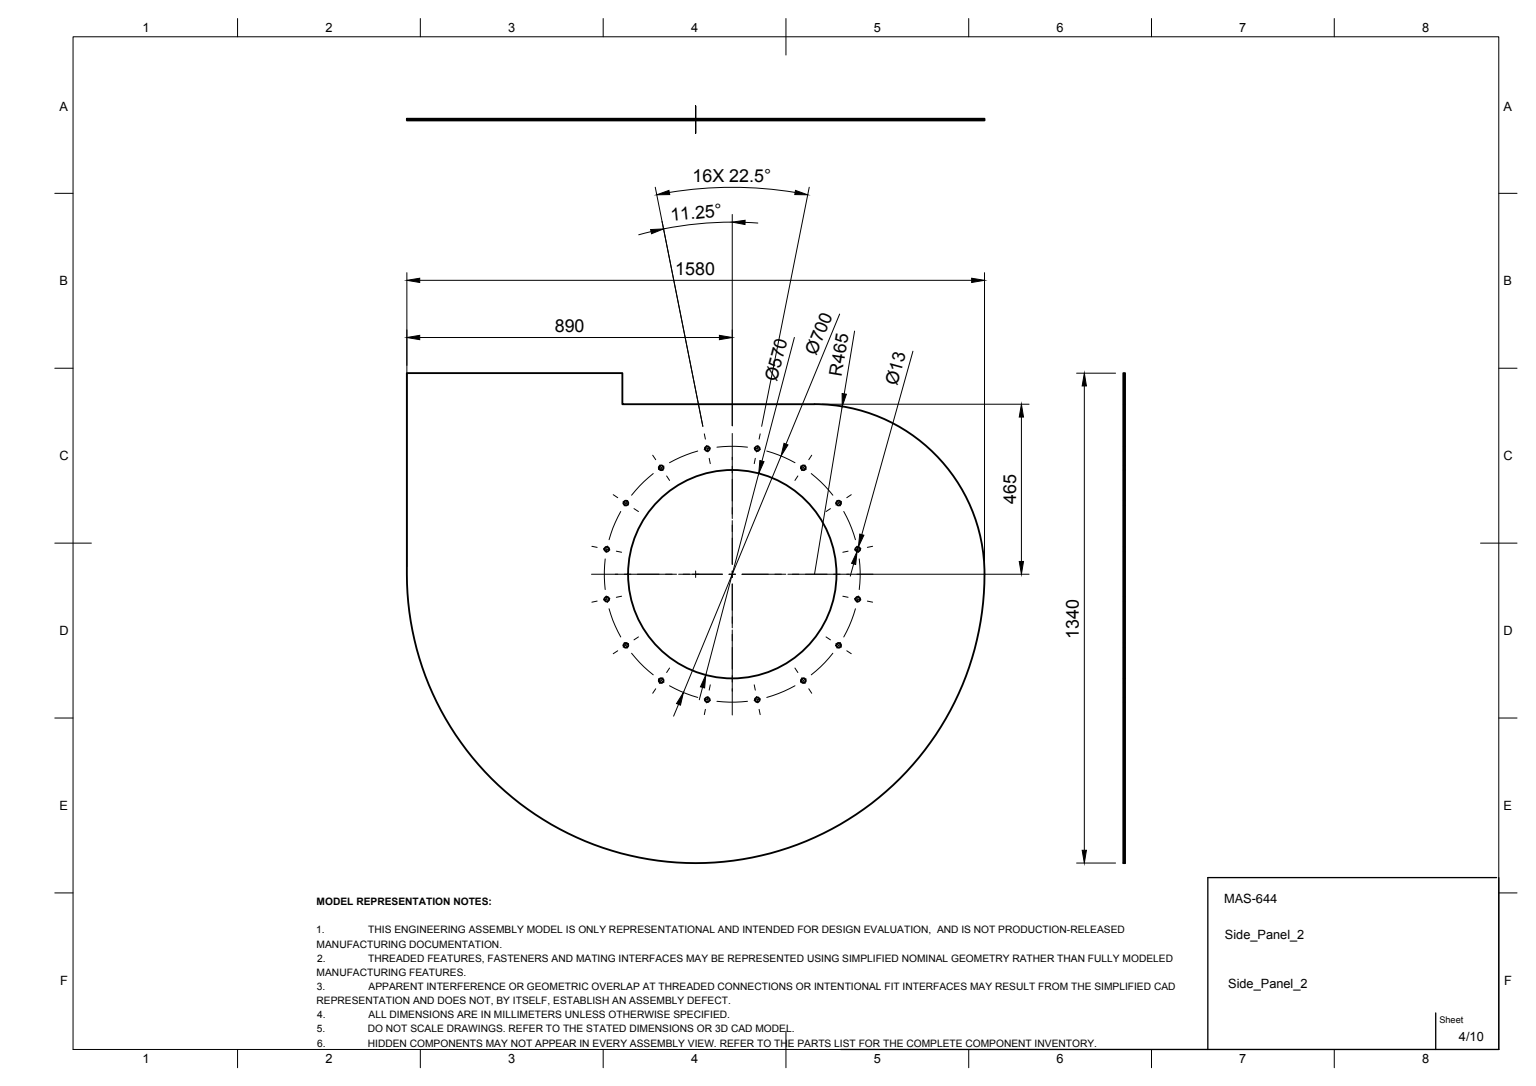
ISO-10303-21;
HEADER;
FILE_DESCRIPTION((''),'2;1');
FILE_NAME('Side_Panel_2.step','2026-10-09T11:38:21-07:00',(''),(''),'','','');
FILE_SCHEMA (('AUTOMOTIVE_DESIGN { 1 0 10303 214 3 1 1 }'));
ENDSEC;
DATA;
#10=MECHANICAL_DESIGN_GEOMETRIC_PRESENTATION_REPRESENTATION('',(#60),#3619);
#44=SHAPE_REPRESENTATION_RELATIONSHIP('SRR','None',#3652,#52) ;
#52=ADVANCED_BREP_SHAPE_REPRESENTATION('',(#68),#3612) ;
#60=STYLED_ITEM('',(#3700),#68) ;
#68=MANIFOLD_SOLID_BREP('Body1',#2084) ;
#77=FACE_BOUND('',#356,.T.) ;
#78=FACE_BOUND('',#357,.T.) ;
#79=FACE_BOUND('',#358,.T.) ;
#80=FACE_BOUND('',#359,.T.) ;
#81=FACE_BOUND('',#360,.T.) ;
#82=FACE_BOUND('',#361,.T.) ;
#83=FACE_BOUND('',#362,.T.) ;
#84=FACE_BOUND('',#363,.T.) ;
#85=FACE_BOUND('',#364,.T.) ;
#86=FACE_BOUND('',#365,.T.) ;
#87=FACE_BOUND('',#366,.T.) ;
#88=FACE_BOUND('',#367,.T.) ;
#89=FACE_BOUND('',#368,.T.) ;
#90=FACE_BOUND('',#369,.T.) ;
#91=FACE_BOUND('',#370,.T.) ;
#92=FACE_BOUND('',#371,.T.) ;
#93=FACE_BOUND('',#372,.T.) ;
#94=FACE_BOUND('',#374,.T.) ;
#95=FACE_BOUND('',#375,.T.) ;
#96=FACE_BOUND('',#376,.T.) ;
#97=FACE_BOUND('',#377,.T.) ;
#98=FACE_BOUND('',#378,.T.) ;
#99=FACE_BOUND('',#379,.T.) ;
#100=FACE_BOUND('',#380,.T.) ;
#101=FACE_BOUND('',#381,.T.) ;
#102=FACE_BOUND('',#382,.T.) ;
#103=FACE_BOUND('',#383,.T.) ;
#104=FACE_BOUND('',#384,.T.) ;
#105=FACE_BOUND('',#385,.T.) ;
#106=FACE_BOUND('',#386,.T.) ;
#107=FACE_BOUND('',#387,.T.) ;
#108=FACE_BOUND('',#388,.T.) ;
#109=FACE_BOUND('',#389,.T.) ;
#110=FACE_BOUND('',#390,.T.) ;
#163=PLANE('',#2249) ;
#164=PLANE('',#2250) ;
#165=PLANE('',#2251) ;
#166=PLANE('',#2252) ;
#167=PLANE('',#2259) ;
#168=PLANE('',#2260) ;
#222=FACE_OUTER_BOUND('',#332,.T.) ;
#223=FACE_OUTER_BOUND('',#333,.T.) ;
#224=FACE_OUTER_BOUND('',#334,.T.) ;
#225=FACE_OUTER_BOUND('',#335,.T.) ;
#226=FACE_OUTER_BOUND('',#336,.T.) ;
#227=FACE_OUTER_BOUND('',#337,.T.) ;
#228=FACE_OUTER_BOUND('',#338,.T.) ;
#229=FACE_OUTER_BOUND('',#339,.T.) ;
#230=FACE_OUTER_BOUND('',#340,.T.) ;
#231=FACE_OUTER_BOUND('',#341,.T.) ;
#232=FACE_OUTER_BOUND('',#342,.T.) ;
#233=FACE_OUTER_BOUND('',#343,.T.) ;
#234=FACE_OUTER_BOUND('',#344,.T.) ;
#235=FACE_OUTER_BOUND('',#345,.T.) ;
#236=FACE_OUTER_BOUND('',#346,.T.) ;
#237=FACE_OUTER_BOUND('',#347,.T.) ;
#238=FACE_OUTER_BOUND('',#348,.T.) ;
#239=FACE_OUTER_BOUND('',#349,.T.) ;
#240=FACE_OUTER_BOUND('',#350,.T.) ;
#241=FACE_OUTER_BOUND('',#351,.T.) ;
#242=FACE_OUTER_BOUND('',#352,.T.) ;
#243=FACE_OUTER_BOUND('',#353,.T.) ;
#244=FACE_OUTER_BOUND('',#354,.T.) ;
#245=FACE_OUTER_BOUND('',#355,.T.) ;
#246=FACE_OUTER_BOUND('',#373,.T.) ;
#332=EDGE_LOOP('',(#1429,#1430,#1431,#1432)) ;
#333=EDGE_LOOP('',(#1433,#1434,#1435,#1436)) ;
#334=EDGE_LOOP('',(#1437,#1438,#1439,#1440)) ;
#335=EDGE_LOOP('',(#1441,#1442,#1443,#1444)) ;
#336=EDGE_LOOP('',(#1445,#1446,#1447,#1448)) ;
#337=EDGE_LOOP('',(#1449,#1450,#1451,#1452)) ;
#338=EDGE_LOOP('',(#1453,#1454,#1455,#1456)) ;
#339=EDGE_LOOP('',(#1457,#1458,#1459,#1460)) ;
#340=EDGE_LOOP('',(#1461,#1462,#1463,#1464)) ;
#341=EDGE_LOOP('',(#1465,#1466,#1467,#1468)) ;
#342=EDGE_LOOP('',(#1469,#1470,#1471,#1472)) ;
#343=EDGE_LOOP('',(#1473,#1474,#1475,#1476)) ;
#344=EDGE_LOOP('',(#1477,#1478,#1479,#1480)) ;
#345=EDGE_LOOP('',(#1481,#1482,#1483,#1484)) ;
#346=EDGE_LOOP('',(#1485,#1486,#1487,#1488)) ;
#347=EDGE_LOOP('',(#1489,#1490,#1491,#1492)) ;
#348=EDGE_LOOP('',(#1493,#1494,#1495,#1496)) ;
#349=EDGE_LOOP('',(#1497,#1498,#1499,#1500)) ;
#350=EDGE_LOOP('',(#1501,#1502,#1503,#1504)) ;
#351=EDGE_LOOP('',(#1505,#1506,#1507,#1508)) ;
#352=EDGE_LOOP('',(#1509,#1510,#1511,#1512)) ;
#353=EDGE_LOOP('',(#1513,#1514,#1515,#1516)) ;
#354=EDGE_LOOP('',(#1517,#1518,#1519,#1520)) ;
#355=EDGE_LOOP('',(#1521,#1522,#1523,#1524,#1525,#1526)) ;
#356=EDGE_LOOP('',(#1527)) ;
#357=EDGE_LOOP('',(#1528)) ;
#358=EDGE_LOOP('',(#1529)) ;
#359=EDGE_LOOP('',(#1530)) ;
#360=EDGE_LOOP('',(#1531)) ;
#361=EDGE_LOOP('',(#1532)) ;
#362=EDGE_LOOP('',(#1533)) ;
#363=EDGE_LOOP('',(#1534)) ;
#364=EDGE_LOOP('',(#1535)) ;
#365=EDGE_LOOP('',(#1536)) ;
#366=EDGE_LOOP('',(#1537)) ;
#367=EDGE_LOOP('',(#1538)) ;
#368=EDGE_LOOP('',(#1539)) ;
#369=EDGE_LOOP('',(#1540)) ;
#370=EDGE_LOOP('',(#1541)) ;
#371=EDGE_LOOP('',(#1542)) ;
#372=EDGE_LOOP('',(#1543)) ;
#373=EDGE_LOOP('',(#1544,#1545,#1546,#1547,#1548,#1549)) ;
#374=EDGE_LOOP('',(#1550)) ;
#375=EDGE_LOOP('',(#1551)) ;
#376=EDGE_LOOP('',(#1552)) ;
#377=EDGE_LOOP('',(#1553)) ;
#378=EDGE_LOOP('',(#1554)) ;
#379=EDGE_LOOP('',(#1555)) ;
#380=EDGE_LOOP('',(#1556)) ;
#381=EDGE_LOOP('',(#1557)) ;
#382=EDGE_LOOP('',(#1558)) ;
#383=EDGE_LOOP('',(#1559)) ;
#384=EDGE_LOOP('',(#1560)) ;
#385=EDGE_LOOP('',(#1561)) ;
#386=EDGE_LOOP('',(#1562)) ;
#387=EDGE_LOOP('',(#1563)) ;
#388=EDGE_LOOP('',(#1564)) ;
#389=EDGE_LOOP('',(#1565)) ;
#390=EDGE_LOOP('',(#1566)) ;
#526=LINE('',#3082,#690) ;
#527=LINE('',#3088,#691) ;
#528=LINE('',#3094,#692) ;
#529=LINE('',#3100,#693) ;
#530=LINE('',#3106,#694) ;
#531=LINE('',#3112,#695) ;
#532=LINE('',#3118,#696) ;
#533=LINE('',#3124,#697) ;
#534=LINE('',#3130,#698) ;
#535=LINE('',#3136,#699) ;
#536=LINE('',#3142,#700) ;
#537=LINE('',#3148,#701) ;
#538=LINE('',#3154,#702) ;
#539=LINE('',#3160,#703) ;
#540=LINE('',#3166,#704) ;
#541=LINE('',#3172,#705) ;
#542=LINE('',#3178,#706) ;
#543=LINE('',#3183,#707) ;
#544=LINE('',#3185,#708) ;
#545=LINE('',#3187,#709) ;
#546=LINE('',#3188,#710) ;
#547=LINE('',#3191,#711) ;
#548=LINE('',#3193,#712) ;
#549=LINE('',#3194,#713) ;
#550=LINE('',#3197,#714) ;
#551=LINE('',#3199,#715) ;
#552=LINE('',#3200,#716) ;
#553=LINE('',#3203,#717) ;
#554=LINE('',#3205,#718) ;
#555=LINE('',#3206,#719) ;
#556=LINE('',#3211,#720) ;
#690=VECTOR('',#2464,6.50000000001752) ;
#691=VECTOR('',#2471,6.50000000000472) ;
#692=VECTOR('',#2478,6.50000000000422) ;
#693=VECTOR('',#2485,6.50000000000406) ;
#694=VECTOR('',#2492,6.50000000000367) ;
#695=VECTOR('',#2499,6.50000000000261) ;
#696=VECTOR('',#2506,6.50000000000162) ;
#697=VECTOR('',#2513,6.50000000000089) ;
#698=VECTOR('',#2520,6.50000000000024) ;
#699=VECTOR('',#2527,6.49999999999945) ;
#700=VECTOR('',#2534,6.49999999999912) ;
#701=VECTOR('',#2541,6.49999999999901) ;
#702=VECTOR('',#2548,6.49999999999912) ;
#703=VECTOR('',#2555,6.49999999999928) ;
#704=VECTOR('',#2562,6.4999999999921) ;
#705=VECTOR('',#2569,6.50000000000001) ;
#706=VECTOR('',#2576,285.) ;
#707=VECTOR('',#2581,1000.) ;
#708=VECTOR('',#2582,1000.) ;
#709=VECTOR('',#2583,1000.) ;
#710=VECTOR('',#2584,1000.) ;
#711=VECTOR('',#2587,1000.) ;
#712=VECTOR('',#2588,1000.) ;
#713=VECTOR('',#2589,1000.) ;
#714=VECTOR('',#2592,1000.) ;
#715=VECTOR('',#2593,1000.) ;
#716=VECTOR('',#2594,1000.) ;
#717=VECTOR('',#2597,1000.) ;
#718=VECTOR('',#2598,1000.) ;
#719=VECTOR('',#2599,1000.) ;
#720=VECTOR('',#2604,1000.) ;
#845=CIRCLE('',#2199,6.50000000001752) ;
#846=CIRCLE('',#2200,6.50000000001752) ;
#847=CIRCLE('',#2202,6.50000000000472) ;
#848=CIRCLE('',#2203,6.50000000000472) ;
#849=CIRCLE('',#2205,6.50000000000422) ;
#850=CIRCLE('',#2206,6.50000000000422) ;
#851=CIRCLE('',#2208,6.50000000000406) ;
#852=CIRCLE('',#2209,6.50000000000406) ;
#853=CIRCLE('',#2211,6.50000000000367) ;
#854=CIRCLE('',#2212,6.50000000000367) ;
#855=CIRCLE('',#2214,6.50000000000261) ;
#856=CIRCLE('',#2215,6.50000000000261) ;
#857=CIRCLE('',#2217,6.50000000000162) ;
#858=CIRCLE('',#2218,6.50000000000162) ;
#859=CIRCLE('',#2220,6.50000000000089) ;
#860=CIRCLE('',#2221,6.50000000000089) ;
#861=CIRCLE('',#2223,6.50000000000024) ;
#862=CIRCLE('',#2224,6.50000000000024) ;
#863=CIRCLE('',#2226,6.49999999999945) ;
#864=CIRCLE('',#2227,6.49999999999945) ;
#865=CIRCLE('',#2229,6.49999999999912) ;
#866=CIRCLE('',#2230,6.49999999999912) ;
#867=CIRCLE('',#2232,6.49999999999901) ;
#868=CIRCLE('',#2233,6.49999999999901) ;
#869=CIRCLE('',#2235,6.49999999999912) ;
#870=CIRCLE('',#2236,6.49999999999912) ;
#871=CIRCLE('',#2238,6.49999999999928) ;
#872=CIRCLE('',#2239,6.49999999999928) ;
#873=CIRCLE('',#2241,6.4999999999921) ;
#874=CIRCLE('',#2242,6.4999999999921) ;
#875=CIRCLE('',#2244,6.50000000000001) ;
#876=CIRCLE('',#2245,6.50000000000001) ;
#877=CIRCLE('',#2247,285.) ;
#878=CIRCLE('',#2248,285.) ;
#879=CIRCLE('',#2254,790.) ;
#880=CIRCLE('',#2255,790.) ;
#881=CIRCLE('',#2257,465.) ;
#882=CIRCLE('',#2258,465.) ;
#957=VERTEX_POINT('',#3079) ;
#958=VERTEX_POINT('',#3081) ;
#959=VERTEX_POINT('',#3085) ;
#960=VERTEX_POINT('',#3087) ;
#961=VERTEX_POINT('',#3091) ;
#962=VERTEX_POINT('',#3093) ;
#963=VERTEX_POINT('',#3097) ;
#964=VERTEX_POINT('',#3099) ;
#965=VERTEX_POINT('',#3103) ;
#966=VERTEX_POINT('',#3105) ;
#967=VERTEX_POINT('',#3109) ;
#968=VERTEX_POINT('',#3111) ;
#969=VERTEX_POINT('',#3115) ;
#970=VERTEX_POINT('',#3117) ;
#971=VERTEX_POINT('',#3121) ;
#972=VERTEX_POINT('',#3123) ;
#973=VERTEX_POINT('',#3127) ;
#974=VERTEX_POINT('',#3129) ;
#975=VERTEX_POINT('',#3133) ;
#976=VERTEX_POINT('',#3135) ;
#977=VERTEX_POINT('',#3139) ;
#978=VERTEX_POINT('',#3141) ;
#979=VERTEX_POINT('',#3145) ;
#980=VERTEX_POINT('',#3147) ;
#981=VERTEX_POINT('',#3151) ;
#982=VERTEX_POINT('',#3153) ;
#983=VERTEX_POINT('',#3157) ;
#984=VERTEX_POINT('',#3159) ;
#985=VERTEX_POINT('',#3163) ;
#986=VERTEX_POINT('',#3165) ;
#987=VERTEX_POINT('',#3169) ;
#988=VERTEX_POINT('',#3171) ;
#989=VERTEX_POINT('',#3175) ;
#990=VERTEX_POINT('',#3177) ;
#991=VERTEX_POINT('',#3181) ;
#992=VERTEX_POINT('',#3182) ;
#993=VERTEX_POINT('',#3184) ;
#994=VERTEX_POINT('',#3186) ;
#995=VERTEX_POINT('',#3190) ;
#996=VERTEX_POINT('',#3192) ;
#997=VERTEX_POINT('',#3196) ;
#998=VERTEX_POINT('',#3198) ;
#999=VERTEX_POINT('',#3202) ;
#1000=VERTEX_POINT('',#3204) ;
#1001=VERTEX_POINT('',#3208) ;
#1002=VERTEX_POINT('',#3210) ;
#1140=EDGE_CURVE('',#957,#957,#845,.T.) ;
#1141=EDGE_CURVE('',#957,#958,#526,.T.) ;
#1142=EDGE_CURVE('',#958,#958,#846,.T.) ;
#1143=EDGE_CURVE('',#959,#959,#847,.T.) ;
#1144=EDGE_CURVE('',#959,#960,#527,.T.) ;
#1145=EDGE_CURVE('',#960,#960,#848,.T.) ;
#1146=EDGE_CURVE('',#961,#961,#849,.T.) ;
#1147=EDGE_CURVE('',#961,#962,#528,.T.) ;
#1148=EDGE_CURVE('',#962,#962,#850,.T.) ;
#1149=EDGE_CURVE('',#963,#963,#851,.T.) ;
#1150=EDGE_CURVE('',#963,#964,#529,.T.) ;
#1151=EDGE_CURVE('',#964,#964,#852,.T.) ;
#1152=EDGE_CURVE('',#965,#965,#853,.T.) ;
#1153=EDGE_CURVE('',#965,#966,#530,.T.) ;
#1154=EDGE_CURVE('',#966,#966,#854,.T.) ;
#1155=EDGE_CURVE('',#967,#967,#855,.T.) ;
#1156=EDGE_CURVE('',#967,#968,#531,.T.) ;
#1157=EDGE_CURVE('',#968,#968,#856,.T.) ;
#1158=EDGE_CURVE('',#969,#969,#857,.T.) ;
#1159=EDGE_CURVE('',#969,#970,#532,.T.) ;
#1160=EDGE_CURVE('',#970,#970,#858,.T.) ;
#1161=EDGE_CURVE('',#971,#971,#859,.T.) ;
#1162=EDGE_CURVE('',#971,#972,#533,.T.) ;
#1163=EDGE_CURVE('',#972,#972,#860,.T.) ;
#1164=EDGE_CURVE('',#973,#973,#861,.T.) ;
#1165=EDGE_CURVE('',#973,#974,#534,.T.) ;
#1166=EDGE_CURVE('',#974,#974,#862,.T.) ;
#1167=EDGE_CURVE('',#975,#975,#863,.T.) ;
#1168=EDGE_CURVE('',#975,#976,#535,.T.) ;
#1169=EDGE_CURVE('',#976,#976,#864,.T.) ;
#1170=EDGE_CURVE('',#977,#977,#865,.T.) ;
#1171=EDGE_CURVE('',#977,#978,#536,.T.) ;
#1172=EDGE_CURVE('',#978,#978,#866,.T.) ;
#1173=EDGE_CURVE('',#979,#979,#867,.T.) ;
#1174=EDGE_CURVE('',#979,#980,#537,.T.) ;
#1175=EDGE_CURVE('',#980,#980,#868,.T.) ;
#1176=EDGE_CURVE('',#981,#981,#869,.T.) ;
#1177=EDGE_CURVE('',#981,#982,#538,.T.) ;
#1178=EDGE_CURVE('',#982,#982,#870,.T.) ;
#1179=EDGE_CURVE('',#983,#983,#871,.T.) ;
#1180=EDGE_CURVE('',#983,#984,#539,.T.) ;
#1181=EDGE_CURVE('',#984,#984,#872,.T.) ;
#1182=EDGE_CURVE('',#985,#985,#873,.T.) ;
#1183=EDGE_CURVE('',#985,#986,#540,.T.) ;
#1184=EDGE_CURVE('',#986,#986,#874,.T.) ;
#1185=EDGE_CURVE('',#987,#987,#875,.T.) ;
#1186=EDGE_CURVE('',#987,#988,#541,.T.) ;
#1187=EDGE_CURVE('',#988,#988,#876,.T.) ;
#1188=EDGE_CURVE('',#989,#989,#877,.T.) ;
#1189=EDGE_CURVE('',#989,#990,#542,.T.) ;
#1190=EDGE_CURVE('',#990,#990,#878,.T.) ;
#1191=EDGE_CURVE('',#991,#992,#543,.T.) ;
#1192=EDGE_CURVE('',#993,#991,#544,.T.) ;
#1193=EDGE_CURVE('',#993,#994,#545,.T.) ;
#1194=EDGE_CURVE('',#994,#992,#546,.T.) ;
#1195=EDGE_CURVE('',#995,#991,#547,.T.) ;
#1196=EDGE_CURVE('',#996,#995,#548,.T.) ;
#1197=EDGE_CURVE('',#996,#993,#549,.T.) ;
#1198=EDGE_CURVE('',#997,#995,#550,.T.) ;
#1199=EDGE_CURVE('',#998,#997,#551,.T.) ;
#1200=EDGE_CURVE('',#998,#996,#552,.T.) ;
#1201=EDGE_CURVE('',#999,#997,#553,.T.) ;
#1202=EDGE_CURVE('',#1000,#999,#554,.T.) ;
#1203=EDGE_CURVE('',#1000,#998,#555,.T.) ;
#1204=EDGE_CURVE('',#1001,#999,#879,.T.) ;
#1205=EDGE_CURVE('',#1002,#1001,#556,.T.) ;
#1206=EDGE_CURVE('',#1002,#1000,#880,.T.) ;
#1207=EDGE_CURVE('',#992,#1001,#881,.T.) ;
#1208=EDGE_CURVE('',#994,#1002,#882,.T.) ;
#1429=ORIENTED_EDGE('',*,*,#1140,.F.) ;
#1430=ORIENTED_EDGE('',*,*,#1141,.T.) ;
#1431=ORIENTED_EDGE('',*,*,#1142,.T.) ;
#1432=ORIENTED_EDGE('',*,*,#1141,.F.) ;
#1433=ORIENTED_EDGE('',*,*,#1143,.F.) ;
#1434=ORIENTED_EDGE('',*,*,#1144,.T.) ;
#1435=ORIENTED_EDGE('',*,*,#1145,.T.) ;
#1436=ORIENTED_EDGE('',*,*,#1144,.F.) ;
#1437=ORIENTED_EDGE('',*,*,#1146,.F.) ;
#1438=ORIENTED_EDGE('',*,*,#1147,.T.) ;
#1439=ORIENTED_EDGE('',*,*,#1148,.T.) ;
#1440=ORIENTED_EDGE('',*,*,#1147,.F.) ;
#1441=ORIENTED_EDGE('',*,*,#1149,.F.) ;
#1442=ORIENTED_EDGE('',*,*,#1150,.T.) ;
#1443=ORIENTED_EDGE('',*,*,#1151,.T.) ;
#1444=ORIENTED_EDGE('',*,*,#1150,.F.) ;
#1445=ORIENTED_EDGE('',*,*,#1152,.F.) ;
#1446=ORIENTED_EDGE('',*,*,#1153,.T.) ;
#1447=ORIENTED_EDGE('',*,*,#1154,.T.) ;
#1448=ORIENTED_EDGE('',*,*,#1153,.F.) ;
#1449=ORIENTED_EDGE('',*,*,#1155,.F.) ;
#1450=ORIENTED_EDGE('',*,*,#1156,.T.) ;
#1451=ORIENTED_EDGE('',*,*,#1157,.T.) ;
#1452=ORIENTED_EDGE('',*,*,#1156,.F.) ;
#1453=ORIENTED_EDGE('',*,*,#1158,.F.) ;
#1454=ORIENTED_EDGE('',*,*,#1159,.T.) ;
#1455=ORIENTED_EDGE('',*,*,#1160,.T.) ;
#1456=ORIENTED_EDGE('',*,*,#1159,.F.) ;
#1457=ORIENTED_EDGE('',*,*,#1161,.F.) ;
#1458=ORIENTED_EDGE('',*,*,#1162,.T.) ;
#1459=ORIENTED_EDGE('',*,*,#1163,.T.) ;
#1460=ORIENTED_EDGE('',*,*,#1162,.F.) ;
#1461=ORIENTED_EDGE('',*,*,#1164,.F.) ;
#1462=ORIENTED_EDGE('',*,*,#1165,.T.) ;
#1463=ORIENTED_EDGE('',*,*,#1166,.T.) ;
#1464=ORIENTED_EDGE('',*,*,#1165,.F.) ;
#1465=ORIENTED_EDGE('',*,*,#1167,.F.) ;
#1466=ORIENTED_EDGE('',*,*,#1168,.T.) ;
#1467=ORIENTED_EDGE('',*,*,#1169,.T.) ;
#1468=ORIENTED_EDGE('',*,*,#1168,.F.) ;
#1469=ORIENTED_EDGE('',*,*,#1170,.F.) ;
#1470=ORIENTED_EDGE('',*,*,#1171,.T.) ;
#1471=ORIENTED_EDGE('',*,*,#1172,.T.) ;
#1472=ORIENTED_EDGE('',*,*,#1171,.F.) ;
#1473=ORIENTED_EDGE('',*,*,#1173,.F.) ;
#1474=ORIENTED_EDGE('',*,*,#1174,.T.) ;
#1475=ORIENTED_EDGE('',*,*,#1175,.T.) ;
#1476=ORIENTED_EDGE('',*,*,#1174,.F.) ;
#1477=ORIENTED_EDGE('',*,*,#1176,.F.) ;
#1478=ORIENTED_EDGE('',*,*,#1177,.T.) ;
#1479=ORIENTED_EDGE('',*,*,#1178,.T.) ;
#1480=ORIENTED_EDGE('',*,*,#1177,.F.) ;
#1481=ORIENTED_EDGE('',*,*,#1179,.F.) ;
#1482=ORIENTED_EDGE('',*,*,#1180,.T.) ;
#1483=ORIENTED_EDGE('',*,*,#1181,.T.) ;
#1484=ORIENTED_EDGE('',*,*,#1180,.F.) ;
#1485=ORIENTED_EDGE('',*,*,#1182,.F.) ;
#1486=ORIENTED_EDGE('',*,*,#1183,.T.) ;
#1487=ORIENTED_EDGE('',*,*,#1184,.T.) ;
#1488=ORIENTED_EDGE('',*,*,#1183,.F.) ;
#1489=ORIENTED_EDGE('',*,*,#1185,.F.) ;
#1490=ORIENTED_EDGE('',*,*,#1186,.T.) ;
#1491=ORIENTED_EDGE('',*,*,#1187,.T.) ;
#1492=ORIENTED_EDGE('',*,*,#1186,.F.) ;
#1493=ORIENTED_EDGE('',*,*,#1188,.F.) ;
#1494=ORIENTED_EDGE('',*,*,#1189,.T.) ;
#1495=ORIENTED_EDGE('',*,*,#1190,.T.) ;
#1496=ORIENTED_EDGE('',*,*,#1189,.F.) ;
#1497=ORIENTED_EDGE('',*,*,#1191,.F.) ;
#1498=ORIENTED_EDGE('',*,*,#1192,.F.) ;
#1499=ORIENTED_EDGE('',*,*,#1193,.T.) ;
#1500=ORIENTED_EDGE('',*,*,#1194,.T.) ;
#1501=ORIENTED_EDGE('',*,*,#1195,.F.) ;
#1502=ORIENTED_EDGE('',*,*,#1196,.F.) ;
#1503=ORIENTED_EDGE('',*,*,#1197,.T.) ;
#1504=ORIENTED_EDGE('',*,*,#1192,.T.) ;
#1505=ORIENTED_EDGE('',*,*,#1198,.F.) ;
#1506=ORIENTED_EDGE('',*,*,#1199,.F.) ;
#1507=ORIENTED_EDGE('',*,*,#1200,.T.) ;
#1508=ORIENTED_EDGE('',*,*,#1196,.T.) ;
#1509=ORIENTED_EDGE('',*,*,#1201,.F.) ;
#1510=ORIENTED_EDGE('',*,*,#1202,.F.) ;
#1511=ORIENTED_EDGE('',*,*,#1203,.T.) ;
#1512=ORIENTED_EDGE('',*,*,#1199,.T.) ;
#1513=ORIENTED_EDGE('',*,*,#1204,.F.) ;
#1514=ORIENTED_EDGE('',*,*,#1205,.F.) ;
#1515=ORIENTED_EDGE('',*,*,#1206,.T.) ;
#1516=ORIENTED_EDGE('',*,*,#1202,.T.) ;
#1517=ORIENTED_EDGE('',*,*,#1207,.F.) ;
#1518=ORIENTED_EDGE('',*,*,#1194,.F.) ;
#1519=ORIENTED_EDGE('',*,*,#1208,.T.) ;
#1520=ORIENTED_EDGE('',*,*,#1205,.T.) ;
#1521=ORIENTED_EDGE('',*,*,#1193,.F.) ;
#1522=ORIENTED_EDGE('',*,*,#1197,.F.) ;
#1523=ORIENTED_EDGE('',*,*,#1200,.F.) ;
#1524=ORIENTED_EDGE('',*,*,#1203,.F.) ;
#1525=ORIENTED_EDGE('',*,*,#1206,.F.) ;
#1526=ORIENTED_EDGE('',*,*,#1208,.F.) ;
#1527=ORIENTED_EDGE('',*,*,#1140,.T.) ;
#1528=ORIENTED_EDGE('',*,*,#1143,.T.) ;
#1529=ORIENTED_EDGE('',*,*,#1146,.T.) ;
#1530=ORIENTED_EDGE('',*,*,#1149,.T.) ;
#1531=ORIENTED_EDGE('',*,*,#1152,.T.) ;
#1532=ORIENTED_EDGE('',*,*,#1155,.T.) ;
#1533=ORIENTED_EDGE('',*,*,#1158,.T.) ;
#1534=ORIENTED_EDGE('',*,*,#1161,.T.) ;
#1535=ORIENTED_EDGE('',*,*,#1164,.T.) ;
#1536=ORIENTED_EDGE('',*,*,#1167,.T.) ;
#1537=ORIENTED_EDGE('',*,*,#1170,.T.) ;
#1538=ORIENTED_EDGE('',*,*,#1173,.T.) ;
#1539=ORIENTED_EDGE('',*,*,#1176,.T.) ;
#1540=ORIENTED_EDGE('',*,*,#1179,.T.) ;
#1541=ORIENTED_EDGE('',*,*,#1182,.T.) ;
#1542=ORIENTED_EDGE('',*,*,#1185,.T.) ;
#1543=ORIENTED_EDGE('',*,*,#1188,.T.) ;
#1544=ORIENTED_EDGE('',*,*,#1191,.T.) ;
#1545=ORIENTED_EDGE('',*,*,#1207,.T.) ;
#1546=ORIENTED_EDGE('',*,*,#1204,.T.) ;
#1547=ORIENTED_EDGE('',*,*,#1201,.T.) ;
#1548=ORIENTED_EDGE('',*,*,#1198,.T.) ;
#1549=ORIENTED_EDGE('',*,*,#1195,.T.) ;
#1550=ORIENTED_EDGE('',*,*,#1142,.F.) ;
#1551=ORIENTED_EDGE('',*,*,#1145,.F.) ;
#1552=ORIENTED_EDGE('',*,*,#1148,.F.) ;
#1553=ORIENTED_EDGE('',*,*,#1151,.F.) ;
#1554=ORIENTED_EDGE('',*,*,#1154,.F.) ;
#1555=ORIENTED_EDGE('',*,*,#1157,.F.) ;
#1556=ORIENTED_EDGE('',*,*,#1160,.F.) ;
#1557=ORIENTED_EDGE('',*,*,#1163,.F.) ;
#1558=ORIENTED_EDGE('',*,*,#1166,.F.) ;
#1559=ORIENTED_EDGE('',*,*,#1169,.F.) ;
#1560=ORIENTED_EDGE('',*,*,#1172,.F.) ;
#1561=ORIENTED_EDGE('',*,*,#1175,.F.) ;
#1562=ORIENTED_EDGE('',*,*,#1178,.F.) ;
#1563=ORIENTED_EDGE('',*,*,#1181,.F.) ;
#1564=ORIENTED_EDGE('',*,*,#1184,.F.) ;
#1565=ORIENTED_EDGE('',*,*,#1187,.F.) ;
#1566=ORIENTED_EDGE('',*,*,#1190,.F.) ;
#1926=CYLINDRICAL_SURFACE('',#2198,6.50000000001752) ;
#1927=CYLINDRICAL_SURFACE('',#2201,6.50000000000472) ;
#1928=CYLINDRICAL_SURFACE('',#2204,6.50000000000422) ;
#1929=CYLINDRICAL_SURFACE('',#2207,6.50000000000406) ;
#1930=CYLINDRICAL_SURFACE('',#2210,6.50000000000367) ;
#1931=CYLINDRICAL_SURFACE('',#2213,6.50000000000261) ;
#1932=CYLINDRICAL_SURFACE('',#2216,6.50000000000162) ;
#1933=CYLINDRICAL_SURFACE('',#2219,6.50000000000089) ;
#1934=CYLINDRICAL_SURFACE('',#2222,6.50000000000024) ;
#1935=CYLINDRICAL_SURFACE('',#2225,6.49999999999945) ;
#1936=CYLINDRICAL_SURFACE('',#2228,6.49999999999912) ;
#1937=CYLINDRICAL_SURFACE('',#2231,6.49999999999901) ;
#1938=CYLINDRICAL_SURFACE('',#2234,6.49999999999912) ;
#1939=CYLINDRICAL_SURFACE('',#2237,6.49999999999928) ;
#1940=CYLINDRICAL_SURFACE('',#2240,6.4999999999921) ;
#1941=CYLINDRICAL_SURFACE('',#2243,6.50000000000001) ;
#1942=CYLINDRICAL_SURFACE('',#2246,285.) ;
#1943=CYLINDRICAL_SURFACE('',#2253,790.) ;
#1944=CYLINDRICAL_SURFACE('',#2256,465.) ;
#1984=ADVANCED_FACE('',(#222),#1926,.F.) ;
#1985=ADVANCED_FACE('',(#223),#1927,.F.) ;
#1986=ADVANCED_FACE('',(#224),#1928,.F.) ;
#1987=ADVANCED_FACE('',(#225),#1929,.F.) ;
#1988=ADVANCED_FACE('',(#226),#1930,.F.) ;
#1989=ADVANCED_FACE('',(#227),#1931,.F.) ;
#1990=ADVANCED_FACE('',(#228),#1932,.F.) ;
#1991=ADVANCED_FACE('',(#229),#1933,.F.) ;
#1992=ADVANCED_FACE('',(#230),#1934,.F.) ;
#1993=ADVANCED_FACE('',(#231),#1935,.F.) ;
#1994=ADVANCED_FACE('',(#232),#1936,.F.) ;
#1995=ADVANCED_FACE('',(#233),#1937,.F.) ;
#1996=ADVANCED_FACE('',(#234),#1938,.F.) ;
#1997=ADVANCED_FACE('',(#235),#1939,.F.) ;
#1998=ADVANCED_FACE('',(#236),#1940,.F.) ;
#1999=ADVANCED_FACE('',(#237),#1941,.F.) ;
#2000=ADVANCED_FACE('',(#238),#1942,.F.) ;
#2001=ADVANCED_FACE('',(#239),#163,.T.) ;
#2002=ADVANCED_FACE('',(#240),#164,.T.) ;
#2003=ADVANCED_FACE('',(#241),#165,.T.) ;
#2004=ADVANCED_FACE('',(#242),#166,.T.) ;
#2005=ADVANCED_FACE('',(#243),#1943,.T.) ;
#2006=ADVANCED_FACE('',(#244),#1944,.T.) ;
#2007=ADVANCED_FACE('',(#245,#77,#78,#79,#80,#81,#82,#83,#84,#85,#86,#87,
#88,#89,#90,#91,#92,#93),#167,.T.) ;
#2008=ADVANCED_FACE('',(#246,#94,#95,#96,#97,#98,#99,#100,#101,#102,#103,
#104,#105,#106,#107,#108,#109,#110),#168,.F.) ;
#2084=CLOSED_SHELL('',(#1984,#1985,#1986,#1987,#1988,#1989,#1990,#1991,
#1992,#1993,#1994,#1995,#1996,#1997,#1998,#1999,#2000,#2001,#2002,#2003,
#2004,#2005,#2006,#2007,#2008)) ;
#2197=AXIS2_PLACEMENT_3D('',#3077,#2458,#2459) ;
#2198=AXIS2_PLACEMENT_3D('',#3078,#2460,#2461) ;
#2199=AXIS2_PLACEMENT_3D('',#3080,#2462,#2463) ;
#2200=AXIS2_PLACEMENT_3D('',#3083,#2465,#2466) ;
#2201=AXIS2_PLACEMENT_3D('',#3084,#2467,#2468) ;
#2202=AXIS2_PLACEMENT_3D('',#3086,#2469,#2470) ;
#2203=AXIS2_PLACEMENT_3D('',#3089,#2472,#2473) ;
#2204=AXIS2_PLACEMENT_3D('',#3090,#2474,#2475) ;
#2205=AXIS2_PLACEMENT_3D('',#3092,#2476,#2477) ;
#2206=AXIS2_PLACEMENT_3D('',#3095,#2479,#2480) ;
#2207=AXIS2_PLACEMENT_3D('',#3096,#2481,#2482) ;
#2208=AXIS2_PLACEMENT_3D('',#3098,#2483,#2484) ;
#2209=AXIS2_PLACEMENT_3D('',#3101,#2486,#2487) ;
#2210=AXIS2_PLACEMENT_3D('',#3102,#2488,#2489) ;
#2211=AXIS2_PLACEMENT_3D('',#3104,#2490,#2491) ;
#2212=AXIS2_PLACEMENT_3D('',#3107,#2493,#2494) ;
#2213=AXIS2_PLACEMENT_3D('',#3108,#2495,#2496) ;
#2214=AXIS2_PLACEMENT_3D('',#3110,#2497,#2498) ;
#2215=AXIS2_PLACEMENT_3D('',#3113,#2500,#2501) ;
#2216=AXIS2_PLACEMENT_3D('',#3114,#2502,#2503) ;
#2217=AXIS2_PLACEMENT_3D('',#3116,#2504,#2505) ;
#2218=AXIS2_PLACEMENT_3D('',#3119,#2507,#2508) ;
#2219=AXIS2_PLACEMENT_3D('',#3120,#2509,#2510) ;
#2220=AXIS2_PLACEMENT_3D('',#3122,#2511,#2512) ;
#2221=AXIS2_PLACEMENT_3D('',#3125,#2514,#2515) ;
#2222=AXIS2_PLACEMENT_3D('',#3126,#2516,#2517) ;
#2223=AXIS2_PLACEMENT_3D('',#3128,#2518,#2519) ;
#2224=AXIS2_PLACEMENT_3D('',#3131,#2521,#2522) ;
#2225=AXIS2_PLACEMENT_3D('',#3132,#2523,#2524) ;
#2226=AXIS2_PLACEMENT_3D('',#3134,#2525,#2526) ;
#2227=AXIS2_PLACEMENT_3D('',#3137,#2528,#2529) ;
#2228=AXIS2_PLACEMENT_3D('',#3138,#2530,#2531) ;
#2229=AXIS2_PLACEMENT_3D('',#3140,#2532,#2533) ;
#2230=AXIS2_PLACEMENT_3D('',#3143,#2535,#2536) ;
#2231=AXIS2_PLACEMENT_3D('',#3144,#2537,#2538) ;
#2232=AXIS2_PLACEMENT_3D('',#3146,#2539,#2540) ;
#2233=AXIS2_PLACEMENT_3D('',#3149,#2542,#2543) ;
#2234=AXIS2_PLACEMENT_3D('',#3150,#2544,#2545) ;
#2235=AXIS2_PLACEMENT_3D('',#3152,#2546,#2547) ;
#2236=AXIS2_PLACEMENT_3D('',#3155,#2549,#2550) ;
#2237=AXIS2_PLACEMENT_3D('',#3156,#2551,#2552) ;
#2238=AXIS2_PLACEMENT_3D('',#3158,#2553,#2554) ;
#2239=AXIS2_PLACEMENT_3D('',#3161,#2556,#2557) ;
#2240=AXIS2_PLACEMENT_3D('',#3162,#2558,#2559) ;
#2241=AXIS2_PLACEMENT_3D('',#3164,#2560,#2561) ;
#2242=AXIS2_PLACEMENT_3D('',#3167,#2563,#2564) ;
#2243=AXIS2_PLACEMENT_3D('',#3168,#2565,#2566) ;
#2244=AXIS2_PLACEMENT_3D('',#3170,#2567,#2568) ;
#2245=AXIS2_PLACEMENT_3D('',#3173,#2570,#2571) ;
#2246=AXIS2_PLACEMENT_3D('',#3174,#2572,#2573) ;
#2247=AXIS2_PLACEMENT_3D('',#3176,#2574,#2575) ;
#2248=AXIS2_PLACEMENT_3D('',#3179,#2577,#2578) ;
#2249=AXIS2_PLACEMENT_3D('',#3180,#2579,#2580) ;
#2250=AXIS2_PLACEMENT_3D('',#3189,#2585,#2586) ;
#2251=AXIS2_PLACEMENT_3D('',#3195,#2590,#2591) ;
#2252=AXIS2_PLACEMENT_3D('',#3201,#2595,#2596) ;
#2253=AXIS2_PLACEMENT_3D('',#3207,#2600,#2601) ;
#2254=AXIS2_PLACEMENT_3D('',#3209,#2602,#2603) ;
#2255=AXIS2_PLACEMENT_3D('',#3212,#2605,#2606) ;
#2256=AXIS2_PLACEMENT_3D('',#3213,#2607,#2608) ;
#2257=AXIS2_PLACEMENT_3D('',#3214,#2609,#2610) ;
#2258=AXIS2_PLACEMENT_3D('',#3215,#2611,#2612) ;
#2259=AXIS2_PLACEMENT_3D('',#3216,#2613,#2614) ;
#2260=AXIS2_PLACEMENT_3D('',#3217,#2615,#2616) ;
#2458=DIRECTION('axis',(0.,0.,1.)) ;
#2459=DIRECTION('refdir',(1.,0.,0.)) ;
#2460=DIRECTION('center_axis',(0.,0.,1.)) ;
#2461=DIRECTION('ref_axis',(1.,0.,0.)) ;
#2462=DIRECTION('center_axis',(0.,0.,1.)) ;
#2463=DIRECTION('ref_axis',(1.,0.,0.)) ;
#2464=DIRECTION('',(0.,0.,1.)) ;
#2465=DIRECTION('center_axis',(0.,0.,1.)) ;
#2466=DIRECTION('ref_axis',(1.,0.,0.)) ;
#2467=DIRECTION('center_axis',(0.,0.,1.)) ;
#2468=DIRECTION('ref_axis',(1.,0.,0.)) ;
#2469=DIRECTION('center_axis',(0.,0.,1.)) ;
#2470=DIRECTION('ref_axis',(1.,0.,0.)) ;
#2471=DIRECTION('',(0.,0.,1.)) ;
#2472=DIRECTION('center_axis',(0.,0.,1.)) ;
#2473=DIRECTION('ref_axis',(1.,0.,0.)) ;
#2474=DIRECTION('center_axis',(0.,0.,1.)) ;
#2475=DIRECTION('ref_axis',(1.,0.,0.)) ;
#2476=DIRECTION('center_axis',(0.,0.,1.)) ;
#2477=DIRECTION('ref_axis',(1.,0.,0.)) ;
#2478=DIRECTION('',(0.,0.,1.)) ;
#2479=DIRECTION('center_axis',(0.,0.,1.)) ;
#2480=DIRECTION('ref_axis',(1.,0.,0.)) ;
#2481=DIRECTION('center_axis',(0.,0.,1.)) ;
#2482=DIRECTION('ref_axis',(1.,0.,0.)) ;
#2483=DIRECTION('center_axis',(0.,0.,1.)) ;
#2484=DIRECTION('ref_axis',(1.,0.,0.)) ;
#2485=DIRECTION('',(0.,0.,1.)) ;
#2486=DIRECTION('center_axis',(0.,0.,1.)) ;
#2487=DIRECTION('ref_axis',(1.,0.,0.)) ;
#2488=DIRECTION('center_axis',(0.,0.,1.)) ;
#2489=DIRECTION('ref_axis',(1.,0.,0.)) ;
#2490=DIRECTION('center_axis',(0.,0.,1.)) ;
#2491=DIRECTION('ref_axis',(1.,0.,0.)) ;
#2492=DIRECTION('',(0.,0.,1.)) ;
#2493=DIRECTION('center_axis',(0.,0.,1.)) ;
#2494=DIRECTION('ref_axis',(1.,0.,0.)) ;
#2495=DIRECTION('center_axis',(0.,0.,1.)) ;
#2496=DIRECTION('ref_axis',(1.,0.,0.)) ;
#2497=DIRECTION('center_axis',(0.,0.,1.)) ;
#2498=DIRECTION('ref_axis',(1.,0.,0.)) ;
#2499=DIRECTION('',(0.,0.,1.)) ;
#2500=DIRECTION('center_axis',(0.,0.,1.)) ;
#2501=DIRECTION('ref_axis',(1.,0.,0.)) ;
#2502=DIRECTION('center_axis',(0.,0.,1.)) ;
#2503=DIRECTION('ref_axis',(1.,0.,0.)) ;
#2504=DIRECTION('center_axis',(0.,0.,1.)) ;
#2505=DIRECTION('ref_axis',(1.,0.,0.)) ;
#2506=DIRECTION('',(0.,0.,1.)) ;
#2507=DIRECTION('center_axis',(0.,0.,1.)) ;
#2508=DIRECTION('ref_axis',(1.,0.,0.)) ;
#2509=DIRECTION('center_axis',(0.,0.,1.)) ;
#2510=DIRECTION('ref_axis',(1.,0.,0.)) ;
#2511=DIRECTION('center_axis',(0.,0.,1.)) ;
#2512=DIRECTION('ref_axis',(1.,0.,0.)) ;
#2513=DIRECTION('',(0.,0.,1.)) ;
#2514=DIRECTION('center_axis',(0.,0.,1.)) ;
#2515=DIRECTION('ref_axis',(1.,0.,0.)) ;
#2516=DIRECTION('center_axis',(0.,0.,1.)) ;
#2517=DIRECTION('ref_axis',(1.,0.,0.)) ;
#2518=DIRECTION('center_axis',(0.,0.,1.)) ;
#2519=DIRECTION('ref_axis',(1.,0.,0.)) ;
#2520=DIRECTION('',(0.,0.,1.)) ;
#2521=DIRECTION('center_axis',(0.,0.,1.)) ;
#2522=DIRECTION('ref_axis',(1.,0.,0.)) ;
#2523=DIRECTION('center_axis',(0.,0.,1.)) ;
#2524=DIRECTION('ref_axis',(1.,0.,0.)) ;
#2525=DIRECTION('center_axis',(0.,0.,1.)) ;
#2526=DIRECTION('ref_axis',(1.,0.,0.)) ;
#2527=DIRECTION('',(0.,0.,1.)) ;
#2528=DIRECTION('center_axis',(0.,0.,1.)) ;
#2529=DIRECTION('ref_axis',(1.,0.,0.)) ;
#2530=DIRECTION('center_axis',(0.,0.,1.)) ;
#2531=DIRECTION('ref_axis',(1.,0.,0.)) ;
#2532=DIRECTION('center_axis',(0.,0.,1.)) ;
#2533=DIRECTION('ref_axis',(1.,0.,0.)) ;
#2534=DIRECTION('',(0.,0.,1.)) ;
#2535=DIRECTION('center_axis',(0.,0.,1.)) ;
#2536=DIRECTION('ref_axis',(1.,0.,0.)) ;
#2537=DIRECTION('center_axis',(0.,0.,1.)) ;
#2538=DIRECTION('ref_axis',(1.,0.,0.)) ;
#2539=DIRECTION('center_axis',(0.,0.,1.)) ;
#2540=DIRECTION('ref_axis',(1.,0.,0.)) ;
#2541=DIRECTION('',(0.,0.,1.)) ;
#2542=DIRECTION('center_axis',(0.,0.,1.)) ;
#2543=DIRECTION('ref_axis',(1.,0.,0.)) ;
#2544=DIRECTION('center_axis',(0.,0.,1.)) ;
#2545=DIRECTION('ref_axis',(1.,0.,0.)) ;
#2546=DIRECTION('center_axis',(0.,0.,1.)) ;
#2547=DIRECTION('ref_axis',(1.,0.,0.)) ;
#2548=DIRECTION('',(0.,0.,1.)) ;
#2549=DIRECTION('center_axis',(0.,0.,1.)) ;
#2550=DIRECTION('ref_axis',(1.,0.,0.)) ;
#2551=DIRECTION('center_axis',(0.,0.,1.)) ;
#2552=DIRECTION('ref_axis',(1.,0.,0.)) ;
#2553=DIRECTION('center_axis',(0.,0.,1.)) ;
#2554=DIRECTION('ref_axis',(1.,0.,0.)) ;
#2555=DIRECTION('',(0.,0.,1.)) ;
#2556=DIRECTION('center_axis',(0.,0.,1.)) ;
#2557=DIRECTION('ref_axis',(1.,0.,0.)) ;
#2558=DIRECTION('center_axis',(0.,0.,1.)) ;
#2559=DIRECTION('ref_axis',(1.,0.,0.)) ;
#2560=DIRECTION('center_axis',(0.,0.,1.)) ;
#2561=DIRECTION('ref_axis',(1.,0.,0.)) ;
#2562=DIRECTION('',(0.,0.,1.)) ;
#2563=DIRECTION('center_axis',(0.,0.,1.)) ;
#2564=DIRECTION('ref_axis',(1.,0.,0.)) ;
#2565=DIRECTION('center_axis',(0.,0.,1.)) ;
#2566=DIRECTION('ref_axis',(1.,0.,0.)) ;
#2567=DIRECTION('center_axis',(0.,0.,1.)) ;
#2568=DIRECTION('ref_axis',(1.,0.,0.)) ;
#2569=DIRECTION('',(0.,0.,1.)) ;
#2570=DIRECTION('center_axis',(0.,0.,1.)) ;
#2571=DIRECTION('ref_axis',(1.,0.,0.)) ;
#2572=DIRECTION('center_axis',(0.,0.,1.)) ;
#2573=DIRECTION('ref_axis',(1.,0.,0.)) ;
#2574=DIRECTION('center_axis',(0.,0.,1.)) ;
#2575=DIRECTION('ref_axis',(1.,0.,0.)) ;
#2576=DIRECTION('',(0.,0.,1.)) ;
#2577=DIRECTION('center_axis',(0.,0.,1.)) ;
#2578=DIRECTION('ref_axis',(1.,0.,0.)) ;
#2579=DIRECTION('center_axis',(0.,1.,0.)) ;
#2580=DIRECTION('ref_axis',(0.,0.,1.)) ;
#2581=DIRECTION('',(-1.,0.,0.)) ;
#2582=DIRECTION('',(0.,0.,1.)) ;
#2583=DIRECTION('',(-1.,-2.46716227694479E-16,0.)) ;
#2584=DIRECTION('',(0.,0.,1.)) ;
#2585=DIRECTION('center_axis',(-1.,1.95921710227969E-15,0.)) ;
#2586=DIRECTION('ref_axis',(-1.95921710227969E-15,-1.,0.)) ;
#2587=DIRECTION('',(-1.95921710227969E-15,-1.,0.)) ;
#2588=DIRECTION('',(0.,0.,1.)) ;
#2589=DIRECTION('',(-1.95921710227969E-15,-1.,0.)) ;
#2590=DIRECTION('center_axis',(0.,1.,0.)) ;
#2591=DIRECTION('ref_axis',(0.,0.,1.)) ;
#2592=DIRECTION('',(-1.,0.,0.)) ;
#2593=DIRECTION('',(0.,0.,1.)) ;
#2594=DIRECTION('',(-1.,0.,0.)) ;
#2595=DIRECTION('center_axis',(1.,0.,0.)) ;
#2596=DIRECTION('ref_axis',(0.,0.,-1.)) ;
#2597=DIRECTION('',(0.,1.,0.)) ;
#2598=DIRECTION('',(0.,0.,1.)) ;
#2599=DIRECTION('',(0.,1.,0.)) ;
#2600=DIRECTION('center_axis',(0.,0.,1.)) ;
#2601=DIRECTION('ref_axis',(1.,0.,0.)) ;
#2602=DIRECTION('center_axis',(0.,0.,1.)) ;
#2603=DIRECTION('ref_axis',(-1.,0.,0.)) ;
#2604=DIRECTION('',(0.,0.,1.)) ;
#2605=DIRECTION('center_axis',(0.,0.,1.)) ;
#2606=DIRECTION('ref_axis',(-1.,0.,0.)) ;
#2607=DIRECTION('center_axis',(0.,0.,1.)) ;
#2608=DIRECTION('ref_axis',(1.,0.,0.)) ;
#2609=DIRECTION('center_axis',(0.,0.,1.)) ;
#2610=DIRECTION('ref_axis',(-1.,0.,0.)) ;
#2611=DIRECTION('center_axis',(0.,0.,1.)) ;
#2612=DIRECTION('ref_axis',(-1.,0.,0.)) ;
#2613=DIRECTION('center_axis',(0.,0.,-1.)) ;
#2614=DIRECTION('ref_axis',(-1.,0.,0.)) ;
#2615=DIRECTION('center_axis',(0.,0.,-1.)) ;
#2616=DIRECTION('ref_axis',(-1.,0.,0.)) ;
#3077=CARTESIAN_POINT('',(0.,0.,0.)) ;
#3078=CARTESIAN_POINT('Origin',(-68.281612705649,343.274848141115,456.5)) ;
#3079=CARTESIAN_POINT('',(-74.7816127056665,343.274848141115,456.5)) ;
#3080=CARTESIAN_POINT('Origin',(-68.281612705649,343.274848141115,456.5)) ;
#3081=CARTESIAN_POINT('',(-74.7816127056665,343.274848141115,461.3)) ;
#3082=CARTESIAN_POINT('',(-74.7816127056665,343.274848141115,456.5)) ;
#3083=CARTESIAN_POINT('Origin',(-68.281612705649,343.274848141115,461.3)) ;
#3084=CARTESIAN_POINT('Origin',(-194.449581556862,291.014364305891,456.5)) ;
#3085=CARTESIAN_POINT('',(-200.949581556867,291.014364305891,456.5)) ;
#3086=CARTESIAN_POINT('Origin',(-194.449581556862,291.014364305891,456.5)) ;
#3087=CARTESIAN_POINT('',(-200.949581556867,291.014364305891,461.3)) ;
#3088=CARTESIAN_POINT('',(-200.949581556867,291.014364305891,456.5)) ;
#3089=CARTESIAN_POINT('Origin',(-194.449581556862,291.014364305891,461.3)) ;
#3090=CARTESIAN_POINT('Origin',(-291.014364305892,194.44958155686,456.5)) ;
#3091=CARTESIAN_POINT('',(-297.514364305897,194.44958155686,456.5)) ;
#3092=CARTESIAN_POINT('Origin',(-291.014364305892,194.44958155686,456.5)) ;
#3093=CARTESIAN_POINT('',(-297.514364305897,194.44958155686,461.3)) ;
#3094=CARTESIAN_POINT('',(-297.514364305896,194.44958155686,456.5)) ;
#3095=CARTESIAN_POINT('Origin',(-291.014364305892,194.44958155686,461.3)) ;
#3096=CARTESIAN_POINT('Origin',(-343.274848141133,68.2816127056437,456.5)) ;
#3097=CARTESIAN_POINT('',(-349.774848141137,68.2816127056437,456.5)) ;
#3098=CARTESIAN_POINT('Origin',(-343.274848141133,68.2816127056437,456.5)) ;
#3099=CARTESIAN_POINT('',(-349.774848141137,68.2816127056437,461.3)) ;
#3100=CARTESIAN_POINT('',(-349.774848141137,68.2816127056437,456.5)) ;
#3101=CARTESIAN_POINT('Origin',(-343.274848141133,68.2816127056437,461.3)) ;
#3102=CARTESIAN_POINT('Origin',(-343.274848141133,-68.2816127056468,456.5)) ;
#3103=CARTESIAN_POINT('',(-349.774848141136,-68.2816127056468,456.5)) ;
#3104=CARTESIAN_POINT('Origin',(-343.274848141133,-68.2816127056468,456.5)) ;
#3105=CARTESIAN_POINT('',(-349.774848141136,-68.2816127056468,461.3)) ;
#3106=CARTESIAN_POINT('',(-349.774848141137,-68.2816127056468,456.5)) ;
#3107=CARTESIAN_POINT('Origin',(-343.274848141133,-68.2816127056468,461.3)) ;
#3108=CARTESIAN_POINT('Origin',(-291.014364305893,-194.449581556863,456.5)) ;
#3109=CARTESIAN_POINT('',(-297.514364305895,-194.449581556863,456.5)) ;
#3110=CARTESIAN_POINT('Origin',(-291.014364305893,-194.449581556863,456.5)) ;
#3111=CARTESIAN_POINT('',(-297.514364305895,-194.449581556863,461.3)) ;
#3112=CARTESIAN_POINT('',(-297.514364305896,-194.449581556863,456.5)) ;
#3113=CARTESIAN_POINT('Origin',(-291.014364305893,-194.449581556863,461.3)) ;
#3114=CARTESIAN_POINT('Origin',(-194.449581556862,-291.014364305894,456.5)) ;
#3115=CARTESIAN_POINT('',(-200.949581556864,-291.014364305894,456.5)) ;
#3116=CARTESIAN_POINT('Origin',(-194.449581556862,-291.014364305894,456.5)) ;
#3117=CARTESIAN_POINT('',(-200.949581556864,-291.014364305894,461.3)) ;
#3118=CARTESIAN_POINT('',(-200.949581556864,-291.014364305894,456.5)) ;
#3119=CARTESIAN_POINT('Origin',(-194.449581556862,-291.014364305894,461.3)) ;
#3120=CARTESIAN_POINT('Origin',(-68.2816127056456,-343.274848141134,456.5)) ;
#3121=CARTESIAN_POINT('',(-74.7816127056465,-343.274848141134,456.5)) ;
#3122=CARTESIAN_POINT('Origin',(-68.2816127056456,-343.274848141134,456.5)) ;
#3123=CARTESIAN_POINT('',(-74.7816127056465,-343.274848141134,461.3)) ;
#3124=CARTESIAN_POINT('',(-74.7816127056465,-343.274848141134,456.5)) ;
#3125=CARTESIAN_POINT('Origin',(-68.2816127056456,-343.274848141134,461.3)) ;
#3126=CARTESIAN_POINT('Origin',(68.2816127056448,-343.274848141134,456.5)) ;
#3127=CARTESIAN_POINT('',(61.7816127056446,-343.274848141134,456.5)) ;
#3128=CARTESIAN_POINT('Origin',(68.2816127056448,-343.274848141134,456.5)) ;
#3129=CARTESIAN_POINT('',(61.7816127056446,-343.274848141134,461.3)) ;
#3130=CARTESIAN_POINT('',(61.7816127056446,-343.274848141134,456.5)) ;
#3131=CARTESIAN_POINT('Origin',(68.2816127056448,-343.274848141134,461.3)) ;
#3132=CARTESIAN_POINT('Origin',(194.449581556861,-291.014364305894,456.5)) ;
#3133=CARTESIAN_POINT('',(187.949581556862,-291.014364305894,456.5)) ;
#3134=CARTESIAN_POINT('Origin',(194.449581556861,-291.014364305894,456.5)) ;
#3135=CARTESIAN_POINT('',(187.949581556862,-291.014364305894,461.3)) ;
#3136=CARTESIAN_POINT('',(187.949581556862,-291.014364305894,456.5)) ;
#3137=CARTESIAN_POINT('Origin',(194.449581556861,-291.014364305894,461.3)) ;
#3138=CARTESIAN_POINT('Origin',(291.014364305892,-194.449581556863,456.5)) ;
#3139=CARTESIAN_POINT('',(284.514364305893,-194.449581556863,456.5)) ;
#3140=CARTESIAN_POINT('Origin',(291.014364305892,-194.449581556863,456.5)) ;
#3141=CARTESIAN_POINT('',(284.514364305893,-194.449581556863,461.3)) ;
#3142=CARTESIAN_POINT('',(284.514364305893,-194.449581556863,456.5)) ;
#3143=CARTESIAN_POINT('Origin',(291.014364305892,-194.449581556863,461.3)) ;
#3144=CARTESIAN_POINT('Origin',(343.274848141132,-68.2816127056467,456.5)) ;
#3145=CARTESIAN_POINT('',(336.774848141133,-68.2816127056467,456.5)) ;
#3146=CARTESIAN_POINT('Origin',(343.274848141132,-68.2816127056467,456.5)) ;
#3147=CARTESIAN_POINT('',(336.774848141133,-68.2816127056467,461.3)) ;
#3148=CARTESIAN_POINT('',(336.774848141133,-68.2816127056467,456.5)) ;
#3149=CARTESIAN_POINT('Origin',(343.274848141132,-68.2816127056467,461.3)) ;
#3150=CARTESIAN_POINT('Origin',(343.274848141132,68.2816127056437,456.5)) ;
#3151=CARTESIAN_POINT('',(336.774848141133,68.2816127056437,456.5)) ;
#3152=CARTESIAN_POINT('Origin',(343.274848141132,68.2816127056437,456.5)) ;
#3153=CARTESIAN_POINT('',(336.774848141133,68.2816127056437,461.3)) ;
#3154=CARTESIAN_POINT('',(336.774848141133,68.2816127056437,456.5)) ;
#3155=CARTESIAN_POINT('Origin',(343.274848141132,68.2816127056437,461.3)) ;
#3156=CARTESIAN_POINT('Origin',(291.014364305892,194.44958155686,456.5)) ;
#3157=CARTESIAN_POINT('',(284.514364305893,194.44958155686,456.5)) ;
#3158=CARTESIAN_POINT('Origin',(291.014364305892,194.44958155686,456.5)) ;
#3159=CARTESIAN_POINT('',(284.514364305893,194.44958155686,461.3)) ;
#3160=CARTESIAN_POINT('',(284.514364305893,194.44958155686,456.5)) ;
#3161=CARTESIAN_POINT('Origin',(291.014364305892,194.44958155686,461.3)) ;
#3162=CARTESIAN_POINT('Origin',(194.44958155687,291.014364305904,456.5)) ;
#3163=CARTESIAN_POINT('',(187.949581556878,291.014364305904,456.5)) ;
#3164=CARTESIAN_POINT('Origin',(194.44958155687,291.014364305904,456.5)) ;
#3165=CARTESIAN_POINT('',(187.949581556878,291.014364305904,461.3)) ;
#3166=CARTESIAN_POINT('',(187.949581556878,291.014364305904,456.5)) ;
#3167=CARTESIAN_POINT('Origin',(194.44958155687,291.014364305904,461.3)) ;
#3168=CARTESIAN_POINT('Origin',(68.2816127056448,343.274848141131,456.5)) ;
#3169=CARTESIAN_POINT('',(61.7816127056448,343.274848141131,456.5)) ;
#3170=CARTESIAN_POINT('Origin',(68.2816127056448,343.274848141131,456.5)) ;
#3171=CARTESIAN_POINT('',(61.7816127056448,343.274848141131,461.3)) ;
#3172=CARTESIAN_POINT('',(61.7816127056448,343.274848141131,456.5)) ;
#3173=CARTESIAN_POINT('Origin',(68.2816127056448,343.274848141131,461.3)) ;
#3174=CARTESIAN_POINT('Origin',(-1.79110198894605E-13,1.12074915713733E-13,
456.5)) ;
#3175=CARTESIAN_POINT('',(-285.,7.71724819380337E-14,456.5)) ;
#3176=CARTESIAN_POINT('Origin',(-1.79110198894605E-13,1.12074915713733E-13,
456.5)) ;
#3177=CARTESIAN_POINT('',(-285.,7.71724819380337E-14,461.3)) ;
#3178=CARTESIAN_POINT('',(-285.,7.71724819380334E-14,456.5)) ;
#3179=CARTESIAN_POINT('Origin',(-1.79110198894605E-13,1.12074915713733E-13,
461.3)) ;
#3180=CARTESIAN_POINT('Origin',(-1.23599047663348E-13,465.,456.5)) ;
#3181=CARTESIAN_POINT('',(300.5,465.,461.3)) ;
#3182=CARTESIAN_POINT('',(-225.,465.,461.3)) ;
#3183=CARTESIAN_POINT('',(-1.23599047663348E-13,465.,461.3)) ;
#3184=CARTESIAN_POINT('',(300.5,465.,456.5)) ;
#3185=CARTESIAN_POINT('',(300.5,465.,456.5)) ;
#3186=CARTESIAN_POINT('',(-225.,465.,456.5)) ;
#3187=CARTESIAN_POINT('',(-225.,465.,456.5)) ;
#3188=CARTESIAN_POINT('',(-225.,465.,456.5)) ;
#3189=CARTESIAN_POINT('Origin',(300.5,465.,456.5)) ;
#3190=CARTESIAN_POINT('',(300.5,550.,461.3)) ;
#3191=CARTESIAN_POINT('',(300.5,465.,461.3)) ;
#3192=CARTESIAN_POINT('',(300.5,550.,456.5)) ;
#3193=CARTESIAN_POINT('',(300.5,550.,456.5)) ;
#3194=CARTESIAN_POINT('',(300.5,465.,456.5)) ;
#3195=CARTESIAN_POINT('Origin',(300.5,550.,456.5)) ;
#3196=CARTESIAN_POINT('',(890.,550.,461.3)) ;
#3197=CARTESIAN_POINT('',(300.5,550.,461.3)) ;
#3198=CARTESIAN_POINT('',(890.,550.,456.5)) ;
#3199=CARTESIAN_POINT('',(890.,550.,456.5)) ;
#3200=CARTESIAN_POINT('',(300.5,550.,456.5)) ;
#3201=CARTESIAN_POINT('Origin',(890.,550.,456.5)) ;
#3202=CARTESIAN_POINT('',(890.,2.23097218176249E-13,461.3)) ;
#3203=CARTESIAN_POINT('',(890.,550.,461.3)) ;
#3204=CARTESIAN_POINT('',(890.,2.23097218176249E-13,456.5)) ;
#3205=CARTESIAN_POINT('',(890.,2.23097218176249E-13,456.5)) ;
#3206=CARTESIAN_POINT('',(890.,550.,456.5)) ;
#3207=CARTESIAN_POINT('Origin',(99.9999999999998,1.12074915713733E-13,456.5)) ;
#3208=CARTESIAN_POINT('',(-690.,1.12074915713733E-13,461.3)) ;
#3209=CARTESIAN_POINT('Origin',(99.9999999999998,1.12074915713733E-13,461.3)) ;
#3210=CARTESIAN_POINT('',(-690.,1.12074915713733E-13,456.5)) ;
#3211=CARTESIAN_POINT('',(-690.,1.12074915713733E-13,456.5)) ;
#3212=CARTESIAN_POINT('Origin',(99.9999999999998,1.12074915713733E-13,456.5)) ;
#3213=CARTESIAN_POINT('Origin',(-225.,1.12074915713733E-13,456.5)) ;
#3214=CARTESIAN_POINT('Origin',(-225.,1.12074915713733E-13,461.3)) ;
#3215=CARTESIAN_POINT('Origin',(-225.,1.12074915713733E-13,456.5)) ;
#3216=CARTESIAN_POINT('Origin',(99.9999999999998,1.12074915713733E-13,456.5)) ;
#3217=CARTESIAN_POINT('Origin',(99.9999999999998,1.12074915713733E-13,461.3)) ;
#3602=UNCERTAINTY_MEASURE_WITH_UNIT(LENGTH_MEASURE(0.01),#3620,
'DISTANCE_ACCURACY_VALUE',
'Maximum model space distance between geometric entities at asserted c
onnectivities') ;
#3609=UNCERTAINTY_MEASURE_WITH_UNIT(LENGTH_MEASURE(0.01),#3620,
'DISTANCE_ACCURACY_VALUE',
'Maximum model space distance between geometric entities at asserted c
onnectivities') ;
#3612=(
GEOMETRIC_REPRESENTATION_CONTEXT(3)
GLOBAL_UNCERTAINTY_ASSIGNED_CONTEXT((#3602))
GLOBAL_UNIT_ASSIGNED_CONTEXT((#3620,#3622,#3623))
REPRESENTATION_CONTEXT('','3D')
) ;
#3619=(
GEOMETRIC_REPRESENTATION_CONTEXT(3)
GLOBAL_UNCERTAINTY_ASSIGNED_CONTEXT((#3609))
GLOBAL_UNIT_ASSIGNED_CONTEXT((#3620,#3622,#3623))
REPRESENTATION_CONTEXT('','3D')
) ;
#3620=(
LENGTH_UNIT()
NAMED_UNIT(*)
SI_UNIT(.MILLI.,.METRE.)
) ;
#3622=(
NAMED_UNIT(*)
PLANE_ANGLE_UNIT()
SI_UNIT($,.RADIAN.)
) ;
#3623=(
NAMED_UNIT(*)
SI_UNIT($,.STERADIAN.)
SOLID_ANGLE_UNIT()
) ;
#3626=SHAPE_DEFINITION_REPRESENTATION(#3635,#3652) ;
#3635=PRODUCT_DEFINITION_SHAPE('',$,#3662) ;
#3652=SHAPE_REPRESENTATION('',(#2197),#3612) ;
#3659=PRODUCT_DEFINITION_CONTEXT('part definition',#3688,'design') ;
#3662=PRODUCT_DEFINITION('Side_Panel_2','Side_Panel_2',#3671,#3659) ;
#3671=PRODUCT_DEFINITION_FORMATION('',$,#3692) ;
#3688=APPLICATION_CONTEXT(
'Core Data for Automotive Mechanical Design Process') ;
#3689=PRODUCT_CONTEXT('part definition',#3688,'mechanical') ;
#3692=PRODUCT('Side_Panel_2','Side_Panel_2',$,(#3689)) ;
#3700=PRESENTATION_STYLE_ASSIGNMENT((#3702)) ;
#3702=SURFACE_STYLE_USAGE(.BOTH.,#3704) ;
#3704=SURFACE_SIDE_STYLE('',(#3706)) ;
#3706=SURFACE_STYLE_FILL_AREA(#3708) ;
#3708=FILL_AREA_STYLE('Opaque(202,209,238)',(#3710)) ;
#3710=FILL_AREA_STYLE_COLOUR('Opaque(202,209,238)',#3712) ;
#3712=COLOUR_RGB('Opaque(202,209,238)', 0.09019608, 0.27058824, 0.51372549) ;
ENDSEC;
END-ISO-10303-21;
